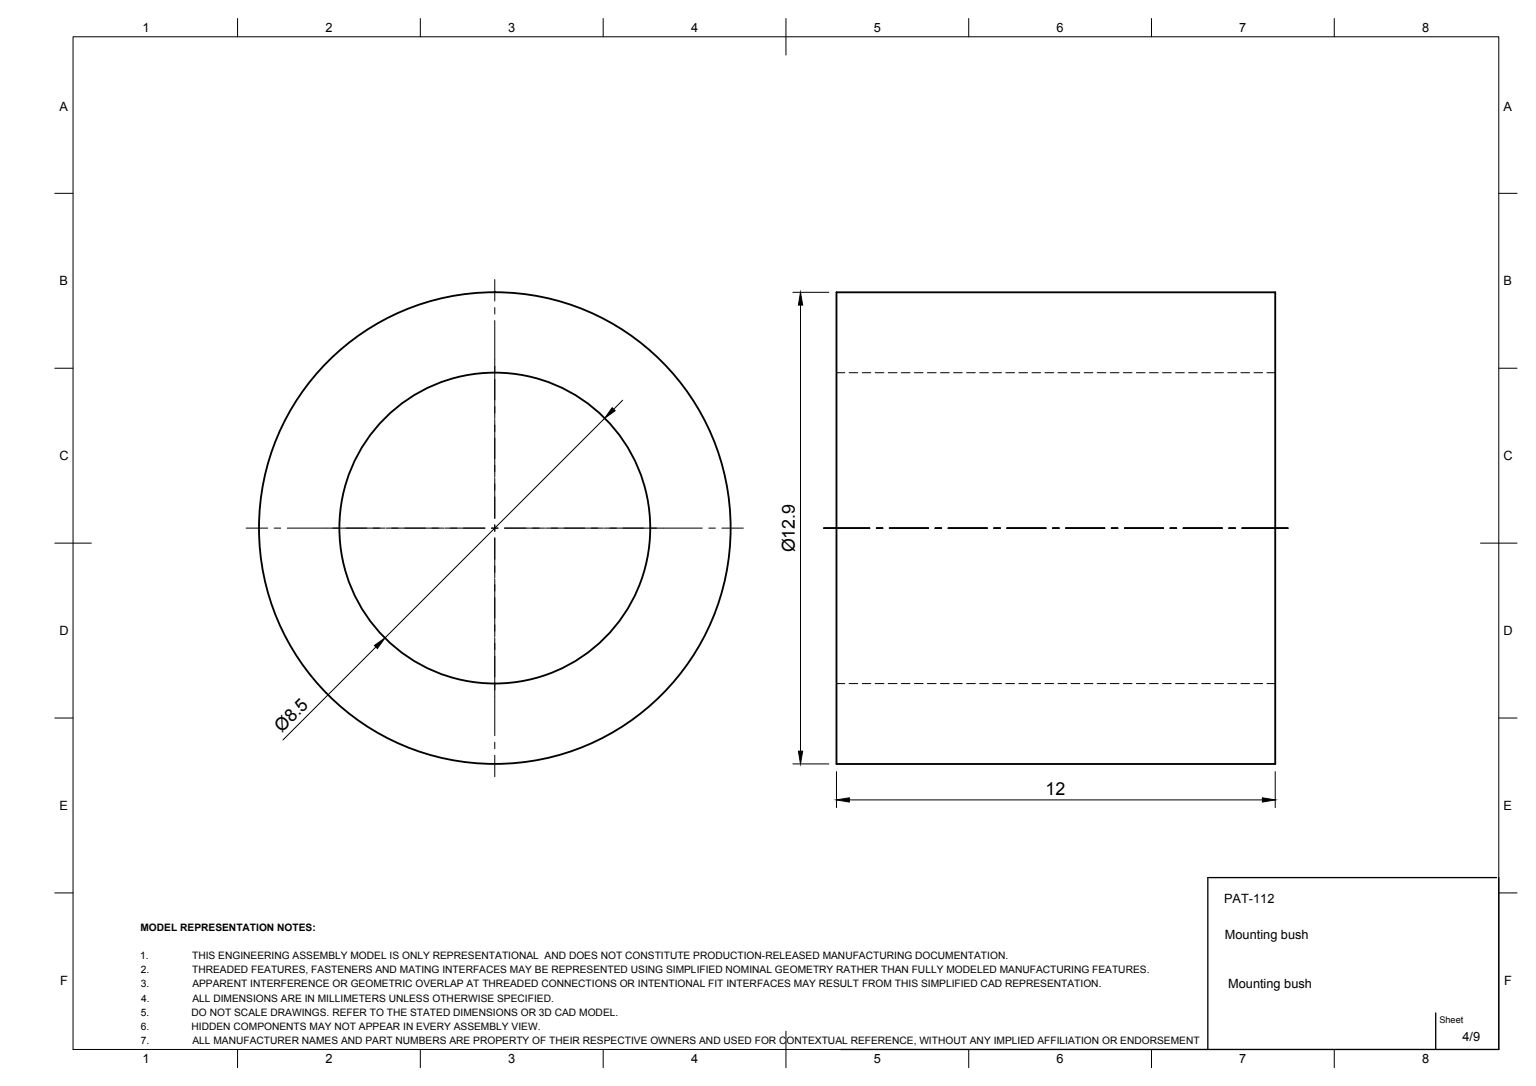
ISO-10303-21;
HEADER;
/* Generated by software containing ST-Developer
 * from STEP Tools, Inc. (www.steptools.com) 
 */

FILE_DESCRIPTION(
/* description */ ('PAT-112'),
/* implementation_level */ '2;1');

FILE_NAME(
/* name */ 'Mounting bush.step',
/* time_stamp */ '2026-11-15T15:25:42-08:00',
/* author */ (''),
/* organization */ (''),
/* preprocessor_version */ 'ST-DEVELOPER v20.2',
/* originating_system */ 'Autodesk Translation Framework v15.17.0.0',
/* authorisation */ '');

FILE_SCHEMA (('AUTOMOTIVE_DESIGN { 1 0 10303 214 3 1 1 }'));
ENDSEC;

DATA;
#10=MECHANICAL_DESIGN_GEOMETRIC_PRESENTATION_REPRESENTATION('',(#109),#2277);
#94=SHAPE_REPRESENTATION_RELATIONSHIP('SRR','None',#2323,#101);
#101=ADVANCED_BREP_SHAPE_REPRESENTATION('',(#117),#2273);
#109=STYLED_ITEM('',(#2370),#117);
#117=MANIFOLD_SOLID_BREP('Body1',#1261);
#141=FACE_BOUND('',#347,.T.);
#142=FACE_BOUND('',#349,.T.);
#180=PLANE('',#1441);
#181=PLANE('',#1442);
#246=FACE_OUTER_BOUND('',#344,.T.);
#247=FACE_OUTER_BOUND('',#345,.T.);
#248=FACE_OUTER_BOUND('',#346,.T.);
#249=FACE_OUTER_BOUND('',#348,.T.);
#344=EDGE_LOOP('',(#1066,#1067,#1068,#1069));
#345=EDGE_LOOP('',(#1070,#1071,#1072,#1073));
#346=EDGE_LOOP('',(#1074));
#347=EDGE_LOOP('',(#1075));
#348=EDGE_LOOP('',(#1076));
#349=EDGE_LOOP('',(#1077));
#443=LINE('',#2138,#538);
#444=LINE('',#2144,#539);
#538=VECTOR('',#1752,0.425);
#539=VECTOR('',#1759,0.645);
#601=CIRCLE('',#1436,0.425);
#602=CIRCLE('',#1437,0.425);
#603=CIRCLE('',#1439,0.645);
#604=CIRCLE('',#1440,0.645);
#689=VERTEX_POINT('',#2135);
#690=VERTEX_POINT('',#2137);
#691=VERTEX_POINT('',#2141);
#692=VERTEX_POINT('',#2143);
#819=EDGE_CURVE('',#689,#689,#601,.T.);
#820=EDGE_CURVE('',#689,#690,#443,.T.);
#821=EDGE_CURVE('',#690,#690,#602,.T.);
#822=EDGE_CURVE('',#691,#691,#603,.T.);
#823=EDGE_CURVE('',#691,#692,#444,.T.);
#824=EDGE_CURVE('',#692,#692,#604,.T.);
#1066=ORIENTED_EDGE('',*,*,#819,.T.);
#1067=ORIENTED_EDGE('',*,*,#820,.T.);
#1068=ORIENTED_EDGE('',*,*,#821,.F.);
#1069=ORIENTED_EDGE('',*,*,#820,.F.);
#1070=ORIENTED_EDGE('',*,*,#822,.F.);
#1071=ORIENTED_EDGE('',*,*,#823,.T.);
#1072=ORIENTED_EDGE('',*,*,#824,.T.);
#1073=ORIENTED_EDGE('',*,*,#823,.F.);
#1074=ORIENTED_EDGE('',*,*,#822,.T.);
#1075=ORIENTED_EDGE('',*,*,#821,.T.);
#1076=ORIENTED_EDGE('',*,*,#824,.F.);
#1077=ORIENTED_EDGE('',*,*,#819,.F.);
#1173=CYLINDRICAL_SURFACE('',#1435,0.425);
#1174=CYLINDRICAL_SURFACE('',#1438,0.645);
#1229=ADVANCED_FACE('',(#246),#1173,.F.);
#1230=ADVANCED_FACE('',(#247),#1174,.T.);
#1231=ADVANCED_FACE('',(#248,#141),#180,.T.);
#1232=ADVANCED_FACE('',(#249,#142),#181,.F.);
#1261=CLOSED_SHELL('',(#1229,#1230,#1231,#1232));
#1434=AXIS2_PLACEMENT_3D('',#2133,#1746,#1747);
#1435=AXIS2_PLACEMENT_3D('',#2134,#1748,#1749);
#1436=AXIS2_PLACEMENT_3D('',#2136,#1750,#1751);
#1437=AXIS2_PLACEMENT_3D('',#2139,#1753,#1754);
#1438=AXIS2_PLACEMENT_3D('',#2140,#1755,#1756);
#1439=AXIS2_PLACEMENT_3D('',#2142,#1757,#1758);
#1440=AXIS2_PLACEMENT_3D('',#2145,#1760,#1761);
#1441=AXIS2_PLACEMENT_3D('',#2146,#1762,#1763);
#1442=AXIS2_PLACEMENT_3D('',#2147,#1764,#1765);
#1746=DIRECTION('axis',(0.,0.,1.));
#1747=DIRECTION('refdir',(1.,0.,0.));
#1748=DIRECTION('center_axis',(0.,0.,1.));
#1749=DIRECTION('ref_axis',(1.,0.,0.));
#1750=DIRECTION('center_axis',(0.,0.,-1.));
#1751=DIRECTION('ref_axis',(1.,0.,0.));
#1752=DIRECTION('',(0.,0.,1.));
#1753=DIRECTION('center_axis',(0.,0.,-1.));
#1754=DIRECTION('ref_axis',(1.,0.,0.));
#1755=DIRECTION('center_axis',(0.,0.,1.));
#1756=DIRECTION('ref_axis',(1.,0.,0.));
#1757=DIRECTION('center_axis',(0.,0.,1.));
#1758=DIRECTION('ref_axis',(1.,0.,0.));
#1759=DIRECTION('',(0.,0.,-1.));
#1760=DIRECTION('center_axis',(0.,0.,1.));
#1761=DIRECTION('ref_axis',(1.,0.,0.));
#1762=DIRECTION('center_axis',(0.,0.,1.));
#1763=DIRECTION('ref_axis',(1.,0.,0.));
#1764=DIRECTION('center_axis',(0.,0.,1.));
#1765=DIRECTION('ref_axis',(1.,0.,0.));
#2133=CARTESIAN_POINT('',(0.,0.,0.));
#2134=CARTESIAN_POINT('Origin',(-4.75,0.,1.2));
#2135=CARTESIAN_POINT('',(-5.175,-5.20474889637625E-17,1.2));
#2136=CARTESIAN_POINT('Origin',(-4.75,0.,1.2));
#2137=CARTESIAN_POINT('',(-5.175,-5.20474889637625E-17,2.4));
#2138=CARTESIAN_POINT('',(-5.175,-5.20474889637625E-17,1.2));
#2139=CARTESIAN_POINT('Origin',(-4.75,0.,2.4));
#2140=CARTESIAN_POINT('Origin',(-4.75,0.,1.2));
#2141=CARTESIAN_POINT('',(-5.395,-7.89897185450042E-17,2.4));
#2142=CARTESIAN_POINT('Origin',(-4.75,0.,2.4));
#2143=CARTESIAN_POINT('',(-5.395,-7.89897185450042E-17,1.2));
#2144=CARTESIAN_POINT('',(-5.395,-7.89897185450043E-17,1.2));
#2145=CARTESIAN_POINT('Origin',(-4.75,0.,1.2));
#2146=CARTESIAN_POINT('Origin',(-4.75,0.,2.4));
#2147=CARTESIAN_POINT('Origin',(-4.75,0.,1.2));
#2263=UNCERTAINTY_MEASURE_WITH_UNIT(LENGTH_MEASURE(0.001),#2278,
'DISTANCE_ACCURACY_VALUE',
'Maximum model space distance between geometric entities at asserted c
onnectivities');
#2267=UNCERTAINTY_MEASURE_WITH_UNIT(LENGTH_MEASURE(0.001),#2278,
'DISTANCE_ACCURACY_VALUE',
'Maximum model space distance between geometric entities at asserted c
onnectivities');
#2273=(
GEOMETRIC_REPRESENTATION_CONTEXT(3)
GLOBAL_UNCERTAINTY_ASSIGNED_CONTEXT((#2263))
GLOBAL_UNIT_ASSIGNED_CONTEXT((#2278,#2280,#2281))
REPRESENTATION_CONTEXT('','3D')
);
#2277=(
GEOMETRIC_REPRESENTATION_CONTEXT(3)
GLOBAL_UNCERTAINTY_ASSIGNED_CONTEXT((#2267))
GLOBAL_UNIT_ASSIGNED_CONTEXT((#2278,#2280,#2281))
REPRESENTATION_CONTEXT('','3D')
);
#2278=(
LENGTH_UNIT()
NAMED_UNIT(*)
SI_UNIT(.CENTI.,.METRE.)
);
#2280=(
NAMED_UNIT(*)
PLANE_ANGLE_UNIT()
SI_UNIT($,.RADIAN.)
);
#2281=(
NAMED_UNIT(*)
SI_UNIT($,.STERADIAN.)
SOLID_ANGLE_UNIT()
);
#2287=SHAPE_DEFINITION_REPRESENTATION(#2298,#2323);
#2298=PRODUCT_DEFINITION_SHAPE('',$,#2333);
#2323=SHAPE_REPRESENTATION('',(#1434),#2273);
#2327=PRODUCT_DEFINITION_CONTEXT('part definition',#2356,'design');
#2333=PRODUCT_DEFINITION('Mounting bush','Mounting bush',#2342,#2327);
#2342=PRODUCT_DEFINITION_FORMATION('',$,#2363);
#2356=APPLICATION_CONTEXT(
'Core Data for Automotive Mechanical Design Process');
#2357=PRODUCT_CONTEXT('part definition',#2356,'mechanical');
#2363=PRODUCT('Mounting bush','Mounting bush','Mounting bush',(#2357));
#2370=PRESENTATION_STYLE_ASSIGNMENT((#2375));
#2375=SURFACE_STYLE_USAGE(.BOTH.,#2380);
#2380=SURFACE_SIDE_STYLE('',(#2385));
#2385=SURFACE_STYLE_FILL_AREA(#2390);
#2390=FILL_AREA_STYLE('Opaque(61,176,222)',(#2395));
#2395=FILL_AREA_STYLE_COLOUR('Opaque(61,176,222)',#2400);
#2400=COLOUR_RGB('Opaque(61,176,222)',0.23921568627451,0.690196078431373,
0.870588235294118);
ENDSEC;
END-ISO-10303-21;
